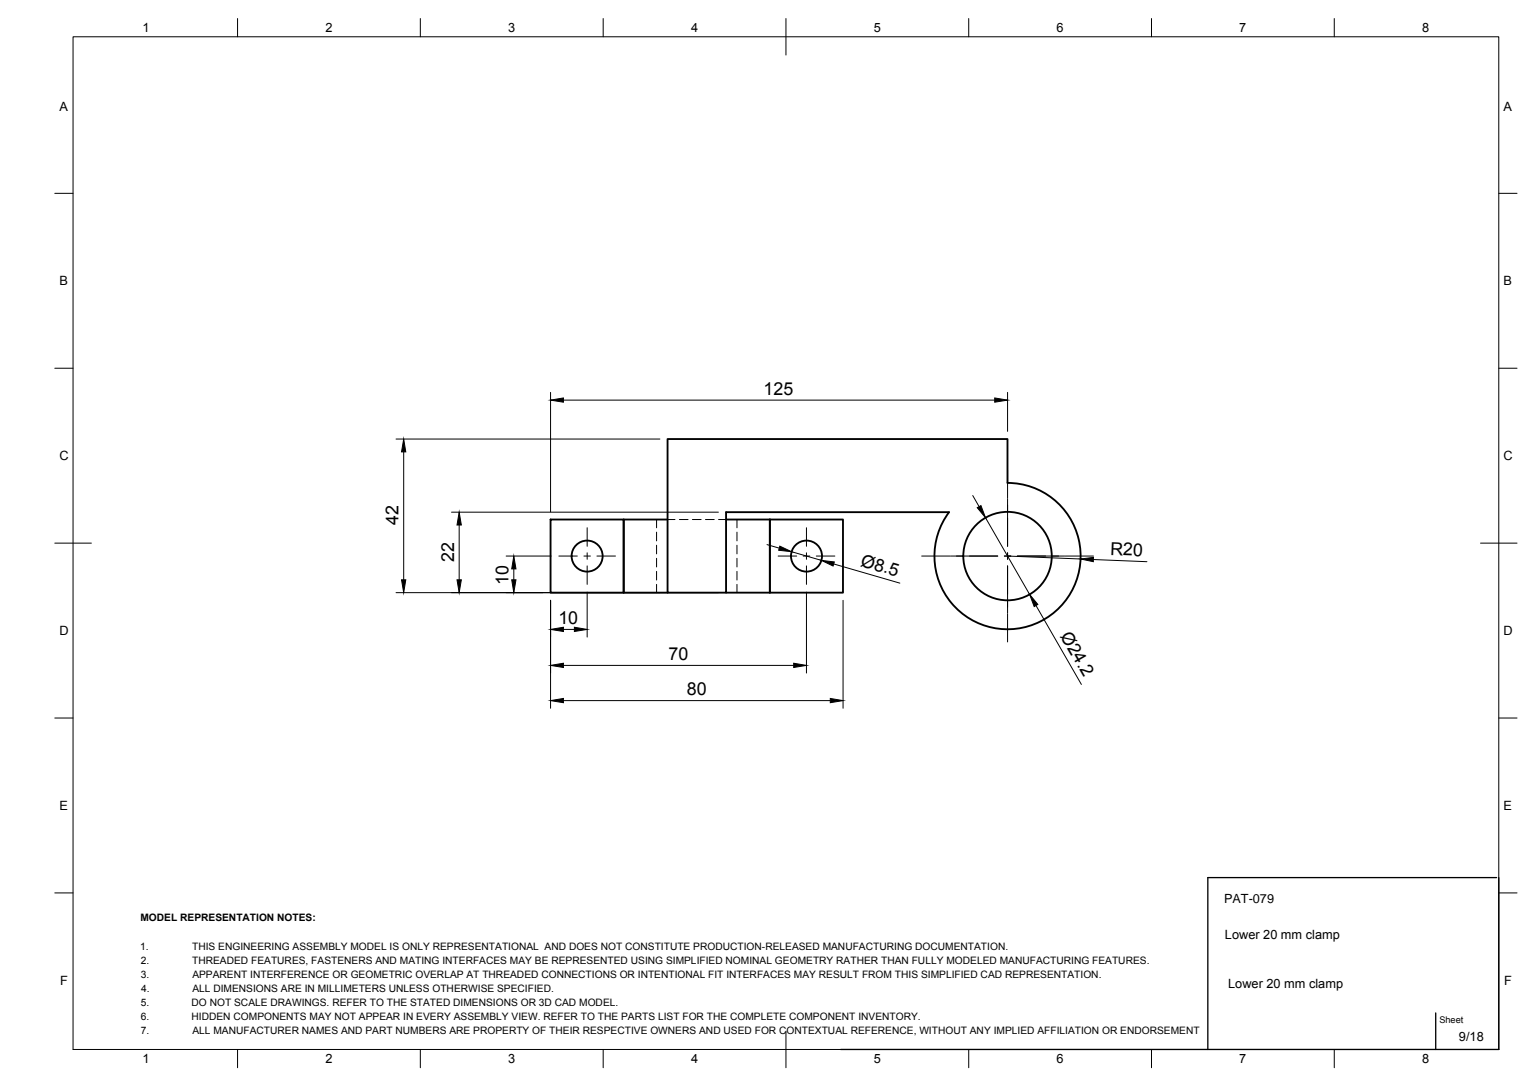
ISO-10303-21;
HEADER;
/* Generated by software containing ST-Developer
 * from STEP Tools, Inc. (www.steptools.com) 
 */

FILE_DESCRIPTION(
/* description */ ('Pipe clamp stand with threaded column'),
/* implementation_level */ '2;1');

FILE_NAME(
/* name */ 'Lower 20 mm clamp.step',
/* time_stamp */ '2026-10-27T10:55:48-07:00',
/* author */ (''),
/* organization */ (''),
/* preprocessor_version */ 'ST-DEVELOPER v20.2',
/* originating_system */ 'Autodesk Translation Framework v15.17.0.0',
/* authorisation */ '');

FILE_SCHEMA (('AUTOMOTIVE_DESIGN { 1 0 10303 214 3 1 1 }'));
ENDSEC;

DATA;
#10=MECHANICAL_DESIGN_GEOMETRIC_PRESENTATION_REPRESENTATION('',(#745,#746,#747),#34433);
#701=SHAPE_REPRESENTATION_RELATIONSHIP('SRR','None',#34543,#723);
#723=ADVANCED_BREP_SHAPE_REPRESENTATION('',(#775,#776,#777),#34411);
#745=STYLED_ITEM('',(#34729),#775);
#746=STYLED_ITEM('',(#34729),#776);
#747=STYLED_ITEM('',(#34729),#777);
#775=MANIFOLD_SOLID_BREP('Body1',#8772);
#776=MANIFOLD_SOLID_BREP('Body2',#8773);
#777=MANIFOLD_SOLID_BREP('Body3',#8774);
#822=FACE_BOUND('',#1783,.T.);
#823=FACE_BOUND('',#1787,.T.);
#824=FACE_BOUND('',#1797,.T.);
#825=FACE_BOUND('',#1800,.T.);
#826=FACE_BOUND('',#1806,.T.);
#827=FACE_BOUND('',#1809,.T.);
#872=PLANE('',#9307);
#873=PLANE('',#9310);
#874=PLANE('',#9317);
#875=PLANE('',#9318);
#876=PLANE('',#9319);
#877=PLANE('',#9320);
#878=PLANE('',#9321);
#879=PLANE('',#9322);
#880=PLANE('',#9323);
#881=PLANE('',#9324);
#882=PLANE('',#9329);
#883=PLANE('',#9333);
#884=PLANE('',#9334);
#885=PLANE('',#9335);
#886=PLANE('',#9336);
#887=PLANE('',#9337);
#888=PLANE('',#9338);
#889=PLANE('',#9342);
#890=PLANE('',#9343);
#891=PLANE('',#9344);
#892=PLANE('',#9345);
#893=PLANE('',#9346);
#894=PLANE('',#9347);
#1266=FACE_OUTER_BOUND('',#1776,.T.);
#1267=FACE_OUTER_BOUND('',#1777,.T.);
#1268=FACE_OUTER_BOUND('',#1778,.T.);
#1269=FACE_OUTER_BOUND('',#1779,.T.);
#1270=FACE_OUTER_BOUND('',#1780,.T.);
#1271=FACE_OUTER_BOUND('',#1781,.T.);
#1272=FACE_OUTER_BOUND('',#1782,.T.);
#1273=FACE_OUTER_BOUND('',#1784,.T.);
#1274=FACE_OUTER_BOUND('',#1785,.T.);
#1275=FACE_OUTER_BOUND('',#1786,.T.);
#1276=FACE_OUTER_BOUND('',#1788,.T.);
#1277=FACE_OUTER_BOUND('',#1789,.T.);
#1278=FACE_OUTER_BOUND('',#1790,.T.);
#1279=FACE_OUTER_BOUND('',#1791,.T.);
#1280=FACE_OUTER_BOUND('',#1792,.T.);
#1281=FACE_OUTER_BOUND('',#1793,.T.);
#1282=FACE_OUTER_BOUND('',#1794,.T.);
#1283=FACE_OUTER_BOUND('',#1795,.T.);
#1284=FACE_OUTER_BOUND('',#1796,.T.);
#1285=FACE_OUTER_BOUND('',#1798,.T.);
#1286=FACE_OUTER_BOUND('',#1799,.T.);
#1287=FACE_OUTER_BOUND('',#1801,.T.);
#1288=FACE_OUTER_BOUND('',#1802,.T.);
#1289=FACE_OUTER_BOUND('',#1803,.T.);
#1290=FACE_OUTER_BOUND('',#1804,.T.);
#1291=FACE_OUTER_BOUND('',#1805,.T.);
#1292=FACE_OUTER_BOUND('',#1807,.T.);
#1293=FACE_OUTER_BOUND('',#1808,.T.);
#1294=FACE_OUTER_BOUND('',#1810,.T.);
#1295=FACE_OUTER_BOUND('',#1811,.T.);
#1776=EDGE_LOOP('',(#6779,#6780,#6781,#6782));
#1777=EDGE_LOOP('',(#6783,#6784,#6785,#6786,#6787,#6788,#6789,#6790));
#1778=EDGE_LOOP('',(#6791,#6792,#6793,#6794));
#1779=EDGE_LOOP('',(#6795,#6796,#6797,#6798));
#1780=EDGE_LOOP('',(#6799,#6800,#6801,#6802));
#1781=EDGE_LOOP('',(#6803,#6804,#6805,#6806));
#1782=EDGE_LOOP('',(#6807,#6808,#6809,#6810,#6811,#6812,#6813));
#1783=EDGE_LOOP('',(#6814));
#1784=EDGE_LOOP('',(#6815,#6816,#6817,#6818));
#1785=EDGE_LOOP('',(#6819,#6820,#6821,#6822));
#1786=EDGE_LOOP('',(#6823,#6824,#6825,#6826,#6827,#6828,#6829));
#1787=EDGE_LOOP('',(#6830));
#1788=EDGE_LOOP('',(#6831,#6832,#6833,#6834,#6835,#6836));
#1789=EDGE_LOOP('',(#6837,#6838,#6839,#6840,#6841,#6842));
#1790=EDGE_LOOP('',(#6843,#6844,#6845,#6846,#6847,#6848,#6849,#6850));
#1791=EDGE_LOOP('',(#6851,#6852,#6853,#6854));
#1792=EDGE_LOOP('',(#6855,#6856,#6857,#6858));
#1793=EDGE_LOOP('',(#6859,#6860,#6861,#6862));
#1794=EDGE_LOOP('',(#6863,#6864,#6865,#6866));
#1795=EDGE_LOOP('',(#6867,#6868,#6869,#6870));
#1796=EDGE_LOOP('',(#6871,#6872,#6873,#6874));
#1797=EDGE_LOOP('',(#6875));
#1798=EDGE_LOOP('',(#6876,#6877,#6878,#6879));
#1799=EDGE_LOOP('',(#6880,#6881,#6882,#6883));
#1800=EDGE_LOOP('',(#6884));
#1801=EDGE_LOOP('',(#6885,#6886,#6887,#6888));
#1802=EDGE_LOOP('',(#6889,#6890,#6891,#6892));
#1803=EDGE_LOOP('',(#6893,#6894,#6895,#6896));
#1804=EDGE_LOOP('',(#6897,#6898,#6899,#6900));
#1805=EDGE_LOOP('',(#6901,#6902,#6903,#6904));
#1806=EDGE_LOOP('',(#6905));
#1807=EDGE_LOOP('',(#6906,#6907,#6908,#6909));
#1808=EDGE_LOOP('',(#6910,#6911,#6912,#6913));
#1809=EDGE_LOOP('',(#6914));
#1810=EDGE_LOOP('',(#6915,#6916,#6917,#6918));
#1811=EDGE_LOOP('',(#6919,#6920,#6921,#6922));
#2291=LINE('',#28038,#2908);
#2292=LINE('',#28041,#2909);
#2293=LINE('',#28044,#2910);
#2294=LINE('',#28048,#2911);
#2295=LINE('',#28050,#2912);
#2296=LINE('',#28052,#2913);
#2297=LINE('',#28055,#2914);
#2298=LINE('',#28058,#2915);
#2299=LINE('',#28059,#2916);
#2300=LINE('',#28064,#2917);
#2301=LINE('',#28069,#2918);
#2302=LINE('',#28073,#2919);
#2303=LINE('',#28077,#2920);
#2304=LINE('',#28079,#2921);
#2305=LINE('',#28080,#2922);
#2306=LINE('',#28083,#2923);
#2307=LINE('',#28085,#2924);
#2308=LINE('',#28087,#2925);
#2309=LINE('',#28089,#2926);
#2310=LINE('',#28090,#2927);
#2311=LINE('',#28093,#2928);
#2312=LINE('',#28094,#2929);
#2313=LINE('',#28097,#2930);
#2314=LINE('',#28098,#2931);
#2315=LINE('',#28100,#2932);
#2316=LINE('',#28101,#2933);
#2317=LINE('',#28104,#2934);
#2318=LINE('',#28105,#2935);
#2319=LINE('',#28108,#2936);
#2320=LINE('',#28109,#2937);
#2321=LINE('',#28112,#2938);
#2322=LINE('',#28117,#2939);
#2323=LINE('',#28123,#2940);
#2324=LINE('',#28128,#2941);
#2325=LINE('',#28130,#2942);
#2326=LINE('',#28132,#2943);
#2327=LINE('',#28133,#2944);
#2328=LINE('',#28136,#2945);
#2329=LINE('',#28138,#2946);
#2330=LINE('',#28139,#2947);
#2331=LINE('',#28142,#2948);
#2332=LINE('',#28144,#2949);
#2333=LINE('',#28145,#2950);
#2334=LINE('',#28147,#2951);
#2335=LINE('',#28148,#2952);
#2336=LINE('',#28155,#2953);
#2337=LINE('',#28160,#2954);
#2338=LINE('',#28162,#2955);
#2339=LINE('',#28164,#2956);
#2340=LINE('',#28165,#2957);
#2341=LINE('',#28168,#2958);
#2342=LINE('',#28170,#2959);
#2343=LINE('',#28171,#2960);
#2344=LINE('',#28174,#2961);
#2345=LINE('',#28176,#2962);
#2346=LINE('',#28177,#2963);
#2347=LINE('',#28179,#2964);
#2348=LINE('',#28180,#2965);
#2908=VECTOR('',#10466,1.);
#2909=VECTOR('',#10469,1.);
#2910=VECTOR('',#10472,1.);
#2911=VECTOR('',#10475,1.);
#2912=VECTOR('',#10476,1.);
#2913=VECTOR('',#10477,1.);
#2914=VECTOR('',#10480,1.);
#2915=VECTOR('',#10483,1.);
#2916=VECTOR('',#10484,1.);
#2917=VECTOR('',#10489,1.21);
#2918=VECTOR('',#10494,1.);
#2919=VECTOR('',#10497,1.);
#2920=VECTOR('',#10502,1.);
#2921=VECTOR('',#10503,1.);
#2922=VECTOR('',#10504,1.);
#2923=VECTOR('',#10507,1.);
#2924=VECTOR('',#10508,1.);
#2925=VECTOR('',#10509,1.);
#2926=VECTOR('',#10510,1.);
#2927=VECTOR('',#10511,1.);
#2928=VECTOR('',#10514,1.);
#2929=VECTOR('',#10515,1.);
#2930=VECTOR('',#10518,1.);
#2931=VECTOR('',#10519,1.);
#2932=VECTOR('',#10522,1.);
#2933=VECTOR('',#10523,1.);
#2934=VECTOR('',#10526,1.);
#2935=VECTOR('',#10527,1.);
#2936=VECTOR('',#10530,1.);
#2937=VECTOR('',#10531,1.);
#2938=VECTOR('',#10534,1.);
#2939=VECTOR('',#10543,1.);
#2940=VECTOR('',#10550,0.425);
#2941=VECTOR('',#10555,1.);
#2942=VECTOR('',#10556,1.);
#2943=VECTOR('',#10557,1.);
#2944=VECTOR('',#10558,1.);
#2945=VECTOR('',#10561,1.);
#2946=VECTOR('',#10562,1.);
#2947=VECTOR('',#10563,1.);
#2948=VECTOR('',#10566,1.);
#2949=VECTOR('',#10567,1.);
#2950=VECTOR('',#10568,1.);
#2951=VECTOR('',#10571,1.);
#2952=VECTOR('',#10572,1.);
#2953=VECTOR('',#10581,0.425);
#2954=VECTOR('',#10586,1.);
#2955=VECTOR('',#10587,1.);
#2956=VECTOR('',#10588,1.);
#2957=VECTOR('',#10589,1.);
#2958=VECTOR('',#10592,1.);
#2959=VECTOR('',#10593,1.);
#2960=VECTOR('',#10594,1.);
#2961=VECTOR('',#10597,1.);
#2962=VECTOR('',#10598,1.);
#2963=VECTOR('',#10599,1.);
#2964=VECTOR('',#10602,1.);
#2965=VECTOR('',#10603,1.);
#3344=CIRCLE('',#9305,1.1);
#3345=CIRCLE('',#9306,1.1);
#3346=CIRCLE('',#9308,2.);
#3347=CIRCLE('',#9309,2.);
#3348=CIRCLE('',#9312,1.21);
#3349=CIRCLE('',#9313,1.21);
#3350=CIRCLE('',#9315,2.);
#3351=CIRCLE('',#9316,2.);
#3352=CIRCLE('',#9325,2.);
#3353=CIRCLE('',#9326,2.);
#3354=CIRCLE('',#9331,0.425);
#3355=CIRCLE('',#9332,0.425);
#3356=CIRCLE('',#9340,0.425);
#3357=CIRCLE('',#9341,0.425);
#3866=VERTEX_POINT('',#28034);
#3867=VERTEX_POINT('',#28035);
#3868=VERTEX_POINT('',#28037);
#3869=VERTEX_POINT('',#28039);
#3870=VERTEX_POINT('',#28043);
#3871=VERTEX_POINT('',#28045);
#3872=VERTEX_POINT('',#28047);
#3873=VERTEX_POINT('',#28049);
#3874=VERTEX_POINT('',#28051);
#3875=VERTEX_POINT('',#28053);
#3876=VERTEX_POINT('',#28057);
#3877=VERTEX_POINT('',#28061);
#3878=VERTEX_POINT('',#28063);
#3879=VERTEX_POINT('',#28067);
#3880=VERTEX_POINT('',#28068);
#3881=VERTEX_POINT('',#28070);
#3882=VERTEX_POINT('',#28072);
#3883=VERTEX_POINT('',#28076);
#3884=VERTEX_POINT('',#28078);
#3885=VERTEX_POINT('',#28082);
#3886=VERTEX_POINT('',#28084);
#3887=VERTEX_POINT('',#28086);
#3888=VERTEX_POINT('',#28088);
#3889=VERTEX_POINT('',#28092);
#3890=VERTEX_POINT('',#28096);
#3891=VERTEX_POINT('',#28103);
#3892=VERTEX_POINT('',#28107);
#3893=VERTEX_POINT('',#28111);
#3894=VERTEX_POINT('',#28120);
#3895=VERTEX_POINT('',#28122);
#3896=VERTEX_POINT('',#28126);
#3897=VERTEX_POINT('',#28127);
#3898=VERTEX_POINT('',#28129);
#3899=VERTEX_POINT('',#28131);
#3900=VERTEX_POINT('',#28135);
#3901=VERTEX_POINT('',#28137);
#3902=VERTEX_POINT('',#28141);
#3903=VERTEX_POINT('',#28143);
#3904=VERTEX_POINT('',#28152);
#3905=VERTEX_POINT('',#28154);
#3906=VERTEX_POINT('',#28158);
#3907=VERTEX_POINT('',#28159);
#3908=VERTEX_POINT('',#28161);
#3909=VERTEX_POINT('',#28163);
#3910=VERTEX_POINT('',#28167);
#3911=VERTEX_POINT('',#28169);
#3912=VERTEX_POINT('',#28173);
#3913=VERTEX_POINT('',#28175);
#4903=EDGE_CURVE('',#3866,#3867,#3344,.T.);
#4904=EDGE_CURVE('',#3868,#3866,#2291,.T.);
#4905=EDGE_CURVE('',#3869,#3868,#3345,.T.);
#4906=EDGE_CURVE('',#3867,#3869,#2292,.T.);
#4907=EDGE_CURVE('',#3868,#3870,#2293,.T.);
#4908=EDGE_CURVE('',#3870,#3871,#3346,.T.);
#4909=EDGE_CURVE('',#3871,#3872,#2294,.T.);
#4910=EDGE_CURVE('',#3872,#3873,#2295,.T.);
#4911=EDGE_CURVE('',#3873,#3874,#2296,.T.);
#4912=EDGE_CURVE('',#3874,#3875,#3347,.T.);
#4913=EDGE_CURVE('',#3875,#3869,#2297,.T.);
#4914=EDGE_CURVE('',#3876,#3866,#2298,.T.);
#4915=EDGE_CURVE('',#3870,#3876,#2299,.T.);
#4916=EDGE_CURVE('',#3877,#3877,#3348,.T.);
#4917=EDGE_CURVE('',#3877,#3878,#2300,.T.);
#4918=EDGE_CURVE('',#3878,#3878,#3349,.T.);
#4919=EDGE_CURVE('',#3879,#3880,#2301,.T.);
#4920=EDGE_CURVE('',#3881,#3879,#3350,.T.);
#4921=EDGE_CURVE('',#3882,#3881,#2302,.T.);
#4922=EDGE_CURVE('',#3882,#3880,#3351,.T.);
#4923=EDGE_CURVE('',#3880,#3883,#2303,.T.);
#4924=EDGE_CURVE('',#3884,#3883,#2304,.T.);
#4925=EDGE_CURVE('',#3884,#3879,#2305,.T.);
#4926=EDGE_CURVE('',#3882,#3885,#2306,.T.);
#4927=EDGE_CURVE('',#3886,#3885,#2307,.T.);
#4928=EDGE_CURVE('',#3887,#3886,#2308,.T.);
#4929=EDGE_CURVE('',#3888,#3887,#2309,.T.);
#4930=EDGE_CURVE('',#3888,#3883,#2310,.T.);
#4931=EDGE_CURVE('',#3881,#3889,#2311,.T.);
#4932=EDGE_CURVE('',#3885,#3889,#2312,.T.);
#4933=EDGE_CURVE('',#3889,#3890,#2313,.T.);
#4934=EDGE_CURVE('',#3890,#3886,#2314,.T.);
#4935=EDGE_CURVE('',#3873,#3884,#2315,.T.);
#4936=EDGE_CURVE('',#3872,#3890,#2316,.T.);
#4937=EDGE_CURVE('',#3891,#3888,#2317,.T.);
#4938=EDGE_CURVE('',#3874,#3891,#2318,.T.);
#4939=EDGE_CURVE('',#3892,#3871,#2319,.T.);
#4940=EDGE_CURVE('',#3887,#3892,#2320,.T.);
#4941=EDGE_CURVE('',#3867,#3893,#2321,.T.);
#4942=EDGE_CURVE('',#3891,#3893,#3352,.T.);
#4943=EDGE_CURVE('',#3876,#3892,#3353,.T.);
#4944=EDGE_CURVE('',#3893,#3875,#2322,.T.);
#4945=EDGE_CURVE('',#3894,#3894,#3354,.T.);
#4946=EDGE_CURVE('',#3894,#3895,#2323,.T.);
#4947=EDGE_CURVE('',#3895,#3895,#3355,.T.);
#4948=EDGE_CURVE('',#3896,#3897,#2324,.T.);
#4949=EDGE_CURVE('',#3896,#3898,#2325,.T.);
#4950=EDGE_CURVE('',#3899,#3898,#2326,.T.);
#4951=EDGE_CURVE('',#3897,#3899,#2327,.T.);
#4952=EDGE_CURVE('',#3897,#3900,#2328,.T.);
#4953=EDGE_CURVE('',#3901,#3899,#2329,.T.);
#4954=EDGE_CURVE('',#3900,#3901,#2330,.T.);
#4955=EDGE_CURVE('',#3900,#3902,#2331,.T.);
#4956=EDGE_CURVE('',#3903,#3901,#2332,.T.);
#4957=EDGE_CURVE('',#3902,#3903,#2333,.T.);
#4958=EDGE_CURVE('',#3902,#3896,#2334,.T.);
#4959=EDGE_CURVE('',#3898,#3903,#2335,.T.);
#4960=EDGE_CURVE('',#3904,#3904,#3356,.T.);
#4961=EDGE_CURVE('',#3904,#3905,#2336,.T.);
#4962=EDGE_CURVE('',#3905,#3905,#3357,.T.);
#4963=EDGE_CURVE('',#3906,#3907,#2337,.T.);
#4964=EDGE_CURVE('',#3906,#3908,#2338,.T.);
#4965=EDGE_CURVE('',#3909,#3908,#2339,.T.);
#4966=EDGE_CURVE('',#3907,#3909,#2340,.T.);
#4967=EDGE_CURVE('',#3907,#3910,#2341,.T.);
#4968=EDGE_CURVE('',#3911,#3909,#2342,.T.);
#4969=EDGE_CURVE('',#3910,#3911,#2343,.T.);
#4970=EDGE_CURVE('',#3910,#3912,#2344,.T.);
#4971=EDGE_CURVE('',#3913,#3911,#2345,.T.);
#4972=EDGE_CURVE('',#3912,#3913,#2346,.T.);
#4973=EDGE_CURVE('',#3912,#3906,#2347,.T.);
#4974=EDGE_CURVE('',#3908,#3913,#2348,.T.);
#6779=ORIENTED_EDGE('',*,*,#4903,.F.);
#6780=ORIENTED_EDGE('',*,*,#4904,.F.);
#6781=ORIENTED_EDGE('',*,*,#4905,.F.);
#6782=ORIENTED_EDGE('',*,*,#4906,.F.);
#6783=ORIENTED_EDGE('',*,*,#4905,.T.);
#6784=ORIENTED_EDGE('',*,*,#4907,.T.);
#6785=ORIENTED_EDGE('',*,*,#4908,.T.);
#6786=ORIENTED_EDGE('',*,*,#4909,.T.);
#6787=ORIENTED_EDGE('',*,*,#4910,.T.);
#6788=ORIENTED_EDGE('',*,*,#4911,.T.);
#6789=ORIENTED_EDGE('',*,*,#4912,.T.);
#6790=ORIENTED_EDGE('',*,*,#4913,.T.);
#6791=ORIENTED_EDGE('',*,*,#4904,.T.);
#6792=ORIENTED_EDGE('',*,*,#4914,.F.);
#6793=ORIENTED_EDGE('',*,*,#4915,.F.);
#6794=ORIENTED_EDGE('',*,*,#4907,.F.);
#6795=ORIENTED_EDGE('',*,*,#4916,.F.);
#6796=ORIENTED_EDGE('',*,*,#4917,.T.);
#6797=ORIENTED_EDGE('',*,*,#4918,.F.);
#6798=ORIENTED_EDGE('',*,*,#4917,.F.);
#6799=ORIENTED_EDGE('',*,*,#4919,.F.);
#6800=ORIENTED_EDGE('',*,*,#4920,.F.);
#6801=ORIENTED_EDGE('',*,*,#4921,.F.);
#6802=ORIENTED_EDGE('',*,*,#4922,.T.);
#6803=ORIENTED_EDGE('',*,*,#4919,.T.);
#6804=ORIENTED_EDGE('',*,*,#4923,.T.);
#6805=ORIENTED_EDGE('',*,*,#4924,.F.);
#6806=ORIENTED_EDGE('',*,*,#4925,.T.);
#6807=ORIENTED_EDGE('',*,*,#4926,.T.);
#6808=ORIENTED_EDGE('',*,*,#4927,.F.);
#6809=ORIENTED_EDGE('',*,*,#4928,.F.);
#6810=ORIENTED_EDGE('',*,*,#4929,.F.);
#6811=ORIENTED_EDGE('',*,*,#4930,.T.);
#6812=ORIENTED_EDGE('',*,*,#4923,.F.);
#6813=ORIENTED_EDGE('',*,*,#4922,.F.);
#6814=ORIENTED_EDGE('',*,*,#4916,.T.);
#6815=ORIENTED_EDGE('',*,*,#4921,.T.);
#6816=ORIENTED_EDGE('',*,*,#4931,.T.);
#6817=ORIENTED_EDGE('',*,*,#4932,.F.);
#6818=ORIENTED_EDGE('',*,*,#4926,.F.);
#6819=ORIENTED_EDGE('',*,*,#4933,.T.);
#6820=ORIENTED_EDGE('',*,*,#4934,.T.);
#6821=ORIENTED_EDGE('',*,*,#4927,.T.);
#6822=ORIENTED_EDGE('',*,*,#4932,.T.);
#6823=ORIENTED_EDGE('',*,*,#4925,.F.);
#6824=ORIENTED_EDGE('',*,*,#4935,.F.);
#6825=ORIENTED_EDGE('',*,*,#4910,.F.);
#6826=ORIENTED_EDGE('',*,*,#4936,.T.);
#6827=ORIENTED_EDGE('',*,*,#4933,.F.);
#6828=ORIENTED_EDGE('',*,*,#4931,.F.);
#6829=ORIENTED_EDGE('',*,*,#4920,.T.);
#6830=ORIENTED_EDGE('',*,*,#4918,.T.);
#6831=ORIENTED_EDGE('',*,*,#4924,.T.);
#6832=ORIENTED_EDGE('',*,*,#4930,.F.);
#6833=ORIENTED_EDGE('',*,*,#4937,.F.);
#6834=ORIENTED_EDGE('',*,*,#4938,.F.);
#6835=ORIENTED_EDGE('',*,*,#4911,.F.);
#6836=ORIENTED_EDGE('',*,*,#4935,.T.);
#6837=ORIENTED_EDGE('',*,*,#4939,.F.);
#6838=ORIENTED_EDGE('',*,*,#4940,.F.);
#6839=ORIENTED_EDGE('',*,*,#4928,.T.);
#6840=ORIENTED_EDGE('',*,*,#4934,.F.);
#6841=ORIENTED_EDGE('',*,*,#4936,.F.);
#6842=ORIENTED_EDGE('',*,*,#4909,.F.);
#6843=ORIENTED_EDGE('',*,*,#4903,.T.);
#6844=ORIENTED_EDGE('',*,*,#4941,.T.);
#6845=ORIENTED_EDGE('',*,*,#4942,.F.);
#6846=ORIENTED_EDGE('',*,*,#4937,.T.);
#6847=ORIENTED_EDGE('',*,*,#4929,.T.);
#6848=ORIENTED_EDGE('',*,*,#4940,.T.);
#6849=ORIENTED_EDGE('',*,*,#4943,.F.);
#6850=ORIENTED_EDGE('',*,*,#4914,.T.);
#6851=ORIENTED_EDGE('',*,*,#4939,.T.);
#6852=ORIENTED_EDGE('',*,*,#4908,.F.);
#6853=ORIENTED_EDGE('',*,*,#4915,.T.);
#6854=ORIENTED_EDGE('',*,*,#4943,.T.);
#6855=ORIENTED_EDGE('',*,*,#4938,.T.);
#6856=ORIENTED_EDGE('',*,*,#4942,.T.);
#6857=ORIENTED_EDGE('',*,*,#4944,.T.);
#6858=ORIENTED_EDGE('',*,*,#4912,.F.);
#6859=ORIENTED_EDGE('',*,*,#4906,.T.);
#6860=ORIENTED_EDGE('',*,*,#4913,.F.);
#6861=ORIENTED_EDGE('',*,*,#4944,.F.);
#6862=ORIENTED_EDGE('',*,*,#4941,.F.);
#6863=ORIENTED_EDGE('',*,*,#4945,.F.);
#6864=ORIENTED_EDGE('',*,*,#4946,.T.);
#6865=ORIENTED_EDGE('',*,*,#4947,.F.);
#6866=ORIENTED_EDGE('',*,*,#4946,.F.);
#6867=ORIENTED_EDGE('',*,*,#4948,.F.);
#6868=ORIENTED_EDGE('',*,*,#4949,.T.);
#6869=ORIENTED_EDGE('',*,*,#4950,.F.);
#6870=ORIENTED_EDGE('',*,*,#4951,.F.);
#6871=ORIENTED_EDGE('',*,*,#4952,.F.);
#6872=ORIENTED_EDGE('',*,*,#4951,.T.);
#6873=ORIENTED_EDGE('',*,*,#4953,.F.);
#6874=ORIENTED_EDGE('',*,*,#4954,.F.);
#6875=ORIENTED_EDGE('',*,*,#4945,.T.);
#6876=ORIENTED_EDGE('',*,*,#4955,.F.);
#6877=ORIENTED_EDGE('',*,*,#4954,.T.);
#6878=ORIENTED_EDGE('',*,*,#4956,.F.);
#6879=ORIENTED_EDGE('',*,*,#4957,.F.);
#6880=ORIENTED_EDGE('',*,*,#4958,.F.);
#6881=ORIENTED_EDGE('',*,*,#4957,.T.);
#6882=ORIENTED_EDGE('',*,*,#4959,.F.);
#6883=ORIENTED_EDGE('',*,*,#4949,.F.);
#6884=ORIENTED_EDGE('',*,*,#4947,.T.);
#6885=ORIENTED_EDGE('',*,*,#4959,.T.);
#6886=ORIENTED_EDGE('',*,*,#4956,.T.);
#6887=ORIENTED_EDGE('',*,*,#4953,.T.);
#6888=ORIENTED_EDGE('',*,*,#4950,.T.);
#6889=ORIENTED_EDGE('',*,*,#4958,.T.);
#6890=ORIENTED_EDGE('',*,*,#4948,.T.);
#6891=ORIENTED_EDGE('',*,*,#4952,.T.);
#6892=ORIENTED_EDGE('',*,*,#4955,.T.);
#6893=ORIENTED_EDGE('',*,*,#4960,.F.);
#6894=ORIENTED_EDGE('',*,*,#4961,.T.);
#6895=ORIENTED_EDGE('',*,*,#4962,.F.);
#6896=ORIENTED_EDGE('',*,*,#4961,.F.);
#6897=ORIENTED_EDGE('',*,*,#4963,.F.);
#6898=ORIENTED_EDGE('',*,*,#4964,.T.);
#6899=ORIENTED_EDGE('',*,*,#4965,.F.);
#6900=ORIENTED_EDGE('',*,*,#4966,.F.);
#6901=ORIENTED_EDGE('',*,*,#4967,.F.);
#6902=ORIENTED_EDGE('',*,*,#4966,.T.);
#6903=ORIENTED_EDGE('',*,*,#4968,.F.);
#6904=ORIENTED_EDGE('',*,*,#4969,.F.);
#6905=ORIENTED_EDGE('',*,*,#4960,.T.);
#6906=ORIENTED_EDGE('',*,*,#4970,.F.);
#6907=ORIENTED_EDGE('',*,*,#4969,.T.);
#6908=ORIENTED_EDGE('',*,*,#4971,.F.);
#6909=ORIENTED_EDGE('',*,*,#4972,.F.);
#6910=ORIENTED_EDGE('',*,*,#4973,.F.);
#6911=ORIENTED_EDGE('',*,*,#4972,.T.);
#6912=ORIENTED_EDGE('',*,*,#4974,.F.);
#6913=ORIENTED_EDGE('',*,*,#4964,.F.);
#6914=ORIENTED_EDGE('',*,*,#4962,.T.);
#6915=ORIENTED_EDGE('',*,*,#4974,.T.);
#6916=ORIENTED_EDGE('',*,*,#4971,.T.);
#6917=ORIENTED_EDGE('',*,*,#4968,.T.);
#6918=ORIENTED_EDGE('',*,*,#4965,.T.);
#6919=ORIENTED_EDGE('',*,*,#4973,.T.);
#6920=ORIENTED_EDGE('',*,*,#4963,.T.);
#6921=ORIENTED_EDGE('',*,*,#4967,.T.);
#6922=ORIENTED_EDGE('',*,*,#4970,.T.);
#8204=CYLINDRICAL_SURFACE('',#9304,1.1);
#8205=CYLINDRICAL_SURFACE('',#9311,1.21);
#8206=CYLINDRICAL_SURFACE('',#9314,2.);
#8207=CYLINDRICAL_SURFACE('',#9327,2.);
#8208=CYLINDRICAL_SURFACE('',#9328,2.);
#8209=CYLINDRICAL_SURFACE('',#9330,0.425);
#8210=CYLINDRICAL_SURFACE('',#9339,0.425);
#8503=ADVANCED_FACE('',(#1266),#8204,.F.);
#8504=ADVANCED_FACE('',(#1267),#872,.T.);
#8505=ADVANCED_FACE('',(#1268),#873,.F.);
#8506=ADVANCED_FACE('',(#1269),#8205,.F.);
#8507=ADVANCED_FACE('',(#1270),#8206,.T.);
#8508=ADVANCED_FACE('',(#1271),#874,.F.);
#8509=ADVANCED_FACE('',(#1272,#822),#875,.T.);
#8510=ADVANCED_FACE('',(#1273),#876,.T.);
#8511=ADVANCED_FACE('',(#1274),#877,.T.);
#8512=ADVANCED_FACE('',(#1275,#823),#878,.T.);
#8513=ADVANCED_FACE('',(#1276),#879,.T.);
#8514=ADVANCED_FACE('',(#1277),#880,.T.);
#8515=ADVANCED_FACE('',(#1278),#881,.F.);
#8516=ADVANCED_FACE('',(#1279),#8207,.T.);
#8517=ADVANCED_FACE('',(#1280),#8208,.T.);
#8518=ADVANCED_FACE('',(#1281),#882,.F.);
#8519=ADVANCED_FACE('',(#1282),#8209,.F.);
#8520=ADVANCED_FACE('',(#1283),#883,.T.);
#8521=ADVANCED_FACE('',(#1284,#824),#884,.T.);
#8522=ADVANCED_FACE('',(#1285),#885,.T.);
#8523=ADVANCED_FACE('',(#1286,#825),#886,.T.);
#8524=ADVANCED_FACE('',(#1287),#887,.T.);
#8525=ADVANCED_FACE('',(#1288),#888,.F.);
#8526=ADVANCED_FACE('',(#1289),#8210,.F.);
#8527=ADVANCED_FACE('',(#1290),#889,.T.);
#8528=ADVANCED_FACE('',(#1291,#826),#890,.T.);
#8529=ADVANCED_FACE('',(#1292),#891,.T.);
#8530=ADVANCED_FACE('',(#1293,#827),#892,.T.);
#8531=ADVANCED_FACE('',(#1294),#893,.T.);
#8532=ADVANCED_FACE('',(#1295),#894,.F.);
#8772=CLOSED_SHELL('',(#8503,#8504,#8505,#8506,#8507,#8508,#8509,#8510,
#8511,#8512,#8513,#8514,#8515,#8516,#8517,#8518));
#8773=CLOSED_SHELL('',(#8519,#8520,#8521,#8522,#8523,#8524,#8525));
#8774=CLOSED_SHELL('',(#8526,#8527,#8528,#8529,#8530,#8531,#8532));
#9303=AXIS2_PLACEMENT_3D('',#28032,#10460,#10461);
#9304=AXIS2_PLACEMENT_3D('',#28033,#10462,#10463);
#9305=AXIS2_PLACEMENT_3D('',#28036,#10464,#10465);
#9306=AXIS2_PLACEMENT_3D('',#28040,#10467,#10468);
#9307=AXIS2_PLACEMENT_3D('',#28042,#10470,#10471);
#9308=AXIS2_PLACEMENT_3D('',#28046,#10473,#10474);
#9309=AXIS2_PLACEMENT_3D('',#28054,#10478,#10479);
#9310=AXIS2_PLACEMENT_3D('',#28056,#10481,#10482);
#9311=AXIS2_PLACEMENT_3D('',#28060,#10485,#10486);
#9312=AXIS2_PLACEMENT_3D('',#28062,#10487,#10488);
#9313=AXIS2_PLACEMENT_3D('',#28065,#10490,#10491);
#9314=AXIS2_PLACEMENT_3D('',#28066,#10492,#10493);
#9315=AXIS2_PLACEMENT_3D('',#28071,#10495,#10496);
#9316=AXIS2_PLACEMENT_3D('',#28074,#10498,#10499);
#9317=AXIS2_PLACEMENT_3D('',#28075,#10500,#10501);
#9318=AXIS2_PLACEMENT_3D('',#28081,#10505,#10506);
#9319=AXIS2_PLACEMENT_3D('',#28091,#10512,#10513);
#9320=AXIS2_PLACEMENT_3D('',#28095,#10516,#10517);
#9321=AXIS2_PLACEMENT_3D('',#28099,#10520,#10521);
#9322=AXIS2_PLACEMENT_3D('',#28102,#10524,#10525);
#9323=AXIS2_PLACEMENT_3D('',#28106,#10528,#10529);
#9324=AXIS2_PLACEMENT_3D('',#28110,#10532,#10533);
#9325=AXIS2_PLACEMENT_3D('',#28113,#10535,#10536);
#9326=AXIS2_PLACEMENT_3D('',#28114,#10537,#10538);
#9327=AXIS2_PLACEMENT_3D('',#28115,#10539,#10540);
#9328=AXIS2_PLACEMENT_3D('',#28116,#10541,#10542);
#9329=AXIS2_PLACEMENT_3D('',#28118,#10544,#10545);
#9330=AXIS2_PLACEMENT_3D('',#28119,#10546,#10547);
#9331=AXIS2_PLACEMENT_3D('',#28121,#10548,#10549);
#9332=AXIS2_PLACEMENT_3D('',#28124,#10551,#10552);
#9333=AXIS2_PLACEMENT_3D('',#28125,#10553,#10554);
#9334=AXIS2_PLACEMENT_3D('',#28134,#10559,#10560);
#9335=AXIS2_PLACEMENT_3D('',#28140,#10564,#10565);
#9336=AXIS2_PLACEMENT_3D('',#28146,#10569,#10570);
#9337=AXIS2_PLACEMENT_3D('',#28149,#10573,#10574);
#9338=AXIS2_PLACEMENT_3D('',#28150,#10575,#10576);
#9339=AXIS2_PLACEMENT_3D('',#28151,#10577,#10578);
#9340=AXIS2_PLACEMENT_3D('',#28153,#10579,#10580);
#9341=AXIS2_PLACEMENT_3D('',#28156,#10582,#10583);
#9342=AXIS2_PLACEMENT_3D('',#28157,#10584,#10585);
#9343=AXIS2_PLACEMENT_3D('',#28166,#10590,#10591);
#9344=AXIS2_PLACEMENT_3D('',#28172,#10595,#10596);
#9345=AXIS2_PLACEMENT_3D('',#28178,#10600,#10601);
#9346=AXIS2_PLACEMENT_3D('',#28181,#10604,#10605);
#9347=AXIS2_PLACEMENT_3D('',#28182,#10606,#10607);
#10460=DIRECTION('axis',(0.,0.,1.));
#10461=DIRECTION('refdir',(1.,0.,0.));
#10462=DIRECTION('center_axis',(0.,1.,0.));
#10463=DIRECTION('ref_axis',(1.,0.,0.));
#10464=DIRECTION('center_axis',(0.,1.,0.));
#10465=DIRECTION('ref_axis',(1.,0.,0.));
#10466=DIRECTION('',(0.,-1.,0.));
#10467=DIRECTION('center_axis',(0.,-1.,0.));
#10468=DIRECTION('ref_axis',(1.,0.,0.));
#10469=DIRECTION('',(0.,1.,0.));
#10470=DIRECTION('center_axis',(0.,1.,0.));
#10471=DIRECTION('ref_axis',(1.,0.,0.));
#10472=DIRECTION('',(1.,0.,0.));
#10473=DIRECTION('center_axis',(0.,1.,0.));
#10474=DIRECTION('ref_axis',(1.,0.,0.));
#10475=DIRECTION('',(0.,0.,1.));
#10476=DIRECTION('',(-1.,0.,0.));
#10477=DIRECTION('',(0.,0.,-1.));
#10478=DIRECTION('center_axis',(0.,1.,0.));
#10479=DIRECTION('ref_axis',(1.,0.,0.));
#10480=DIRECTION('',(1.,0.,0.));
#10481=DIRECTION('center_axis',(0.,0.,-1.));
#10482=DIRECTION('ref_axis',(-1.,0.,0.));
#10483=DIRECTION('',(-1.,0.,0.));
#10484=DIRECTION('',(0.,-1.,0.));
#10485=DIRECTION('center_axis',(0.,0.,1.));
#10486=DIRECTION('ref_axis',(1.,0.,0.));
#10487=DIRECTION('center_axis',(0.,0.,1.));
#10488=DIRECTION('ref_axis',(1.,0.,0.));
#10489=DIRECTION('',(0.,0.,1.));
#10490=DIRECTION('center_axis',(0.,0.,-1.));
#10491=DIRECTION('ref_axis',(1.,0.,0.));
#10492=DIRECTION('center_axis',(0.,0.,1.));
#10493=DIRECTION('ref_axis',(-0.447213595499958,-0.894427190999916,0.));
#10494=DIRECTION('',(0.,0.,-1.));
#10495=DIRECTION('center_axis',(0.,0.,1.));
#10496=DIRECTION('ref_axis',(1.,0.,0.));
#10497=DIRECTION('',(0.,0.,1.));
#10498=DIRECTION('center_axis',(0.,0.,1.));
#10499=DIRECTION('ref_axis',(1.,0.,0.));
#10500=DIRECTION('center_axis',(0.,1.,0.));
#10501=DIRECTION('ref_axis',(1.,0.,0.));
#10502=DIRECTION('',(1.,0.,0.));
#10503=DIRECTION('',(0.,0.,-1.));
#10504=DIRECTION('',(-1.,0.,0.));
#10505=DIRECTION('center_axis',(0.,0.,-1.));
#10506=DIRECTION('ref_axis',(-1.,0.,0.));
#10507=DIRECTION('',(0.,1.,0.));
#10508=DIRECTION('',(-1.,0.,0.));
#10509=DIRECTION('',(0.,1.,0.));
#10510=DIRECTION('',(1.,0.,0.));
#10511=DIRECTION('',(0.,1.,0.));
#10512=DIRECTION('center_axis',(-1.,0.,0.));
#10513=DIRECTION('ref_axis',(0.,0.,1.));
#10514=DIRECTION('',(0.,1.,0.));
#10515=DIRECTION('',(0.,0.,1.));
#10516=DIRECTION('center_axis',(0.,1.,0.));
#10517=DIRECTION('ref_axis',(0.,0.,1.));
#10518=DIRECTION('',(1.,0.,0.));
#10519=DIRECTION('',(0.,0.,-1.));
#10520=DIRECTION('center_axis',(0.,0.,1.));
#10521=DIRECTION('ref_axis',(1.,0.,0.));
#10522=DIRECTION('',(0.,1.,0.));
#10523=DIRECTION('',(0.,1.,0.));
#10524=DIRECTION('center_axis',(-1.,0.,0.));
#10525=DIRECTION('ref_axis',(0.,0.,1.));
#10526=DIRECTION('',(0.,0.,-1.));
#10527=DIRECTION('',(0.,-1.,0.));
#10528=DIRECTION('center_axis',(1.,0.,0.));
#10529=DIRECTION('ref_axis',(0.,0.,-1.));
#10530=DIRECTION('',(0.,1.,0.));
#10531=DIRECTION('',(0.,0.,1.));
#10532=DIRECTION('center_axis',(0.,1.,0.));
#10533=DIRECTION('ref_axis',(1.,0.,0.));
#10534=DIRECTION('',(-1.,0.,0.));
#10535=DIRECTION('center_axis',(0.,1.,0.));
#10536=DIRECTION('ref_axis',(1.,0.,0.));
#10537=DIRECTION('center_axis',(0.,1.,0.));
#10538=DIRECTION('ref_axis',(1.,0.,0.));
#10539=DIRECTION('center_axis',(0.,1.,0.));
#10540=DIRECTION('ref_axis',(1.,0.,0.));
#10541=DIRECTION('center_axis',(0.,1.,0.));
#10542=DIRECTION('ref_axis',(1.,0.,0.));
#10543=DIRECTION('',(0.,1.,0.));
#10544=DIRECTION('center_axis',(0.,0.,-1.));
#10545=DIRECTION('ref_axis',(-1.,0.,0.));
#10546=DIRECTION('center_axis',(0.,0.,1.));
#10547=DIRECTION('ref_axis',(1.,0.,0.));
#10548=DIRECTION('center_axis',(0.,0.,1.));
#10549=DIRECTION('ref_axis',(1.,0.,0.));
#10550=DIRECTION('',(0.,0.,1.));
#10551=DIRECTION('center_axis',(0.,0.,-1.));
#10552=DIRECTION('ref_axis',(1.,0.,0.));
#10553=DIRECTION('center_axis',(-1.,0.,0.));
#10554=DIRECTION('ref_axis',(0.,0.,1.));
#10555=DIRECTION('',(0.,0.,-1.));
#10556=DIRECTION('',(0.,1.,0.));
#10557=DIRECTION('',(0.,0.,1.));
#10558=DIRECTION('',(0.,1.,0.));
#10559=DIRECTION('center_axis',(0.,0.,-1.));
#10560=DIRECTION('ref_axis',(-1.,0.,0.));
#10561=DIRECTION('',(1.,0.,0.));
#10562=DIRECTION('',(-1.,0.,0.));
#10563=DIRECTION('',(0.,1.,0.));
#10564=DIRECTION('center_axis',(1.,0.,0.));
#10565=DIRECTION('ref_axis',(0.,0.,-1.));
#10566=DIRECTION('',(0.,0.,1.));
#10567=DIRECTION('',(0.,0.,-1.));
#10568=DIRECTION('',(0.,1.,0.));
#10569=DIRECTION('center_axis',(0.,0.,1.));
#10570=DIRECTION('ref_axis',(1.,0.,0.));
#10571=DIRECTION('',(-1.,0.,0.));
#10572=DIRECTION('',(1.,0.,0.));
#10573=DIRECTION('center_axis',(0.,1.,0.));
#10574=DIRECTION('ref_axis',(0.,0.,1.));
#10575=DIRECTION('center_axis',(0.,1.,0.));
#10576=DIRECTION('ref_axis',(1.,0.,0.));
#10577=DIRECTION('center_axis',(0.,0.,1.));
#10578=DIRECTION('ref_axis',(1.,0.,0.));
#10579=DIRECTION('center_axis',(0.,0.,1.));
#10580=DIRECTION('ref_axis',(1.,0.,0.));
#10581=DIRECTION('',(0.,0.,1.));
#10582=DIRECTION('center_axis',(0.,0.,-1.));
#10583=DIRECTION('ref_axis',(1.,0.,0.));
#10584=DIRECTION('center_axis',(-1.,0.,0.));
#10585=DIRECTION('ref_axis',(0.,0.,1.));
#10586=DIRECTION('',(0.,0.,-1.));
#10587=DIRECTION('',(0.,1.,0.));
#10588=DIRECTION('',(0.,0.,1.));
#10589=DIRECTION('',(0.,1.,0.));
#10590=DIRECTION('center_axis',(0.,0.,-1.));
#10591=DIRECTION('ref_axis',(-1.,0.,0.));
#10592=DIRECTION('',(1.,0.,0.));
#10593=DIRECTION('',(-1.,0.,0.));
#10594=DIRECTION('',(0.,1.,0.));
#10595=DIRECTION('center_axis',(1.,0.,0.));
#10596=DIRECTION('ref_axis',(0.,0.,-1.));
#10597=DIRECTION('',(0.,0.,1.));
#10598=DIRECTION('',(0.,0.,-1.));
#10599=DIRECTION('',(0.,1.,0.));
#10600=DIRECTION('center_axis',(0.,0.,1.));
#10601=DIRECTION('ref_axis',(1.,0.,0.));
#10602=DIRECTION('',(-1.,0.,0.));
#10603=DIRECTION('',(1.,0.,0.));
#10604=DIRECTION('center_axis',(0.,1.,0.));
#10605=DIRECTION('ref_axis',(0.,0.,1.));
#10606=DIRECTION('center_axis',(0.,1.,0.));
#10607=DIRECTION('ref_axis',(1.,0.,0.));
#28032=CARTESIAN_POINT('',(0.,0.,0.));
#28033=CARTESIAN_POINT('Origin',(0.,-1.1,18.));
#28034=CARTESIAN_POINT('',(1.09971587239614,-1.,17.975));
#28035=CARTESIAN_POINT('',(-1.09971587239614,-1.,17.975));
#28036=CARTESIAN_POINT('Origin',(0.,-1.,18.));
#28037=CARTESIAN_POINT('',(1.09971587239614,1.,17.975));
#28038=CARTESIAN_POINT('',(1.09971587239614,-1.1,17.975));
#28039=CARTESIAN_POINT('',(-1.09971587239614,1.,17.975));
#28040=CARTESIAN_POINT('Origin',(0.,1.,18.));
#28041=CARTESIAN_POINT('',(-1.09971587239614,-1.1,17.975));
#28042=CARTESIAN_POINT('Origin',(0.,1.,18.));
#28043=CARTESIAN_POINT('',(1.99984374389601,1.,17.975));
#28044=CARTESIAN_POINT('',(2.,1.,17.975));
#28045=CARTESIAN_POINT('',(0.8,1.,16.1669697220177));
#28046=CARTESIAN_POINT('Origin',(0.,1.,18.));
#28047=CARTESIAN_POINT('',(0.8,1.,16.2));
#28048=CARTESIAN_POINT('',(0.8,1.,17.1));
#28049=CARTESIAN_POINT('',(-0.8,1.,16.2));
#28050=CARTESIAN_POINT('',(-0.4,1.,16.2));
#28051=CARTESIAN_POINT('',(-0.8,1.,16.1669697220177));
#28052=CARTESIAN_POINT('',(-0.8,1.,16.5));
#28053=CARTESIAN_POINT('',(-1.99984374389601,1.,17.975));
#28054=CARTESIAN_POINT('Origin',(0.,1.,18.));
#28055=CARTESIAN_POINT('',(2.,1.,17.975));
#28056=CARTESIAN_POINT('Origin',(4.,-1.1,17.975));
#28057=CARTESIAN_POINT('',(1.99984374389601,-1.,17.975));
#28058=CARTESIAN_POINT('',(2.,-1.,17.975));
#28059=CARTESIAN_POINT('',(1.99984374389601,-1.,17.975));
#28060=CARTESIAN_POINT('Origin',(-8.5,0.,14.9));
#28061=CARTESIAN_POINT('',(-9.71,-1.4818226269683E-16,15.));
#28062=CARTESIAN_POINT('Origin',(-8.5,0.,15.));
#28063=CARTESIAN_POINT('',(-9.71,1.4818226269683E-16,16.2));
#28064=CARTESIAN_POINT('',(-9.71,-1.4818226269683E-16,14.9));
#28065=CARTESIAN_POINT('Origin',(-8.5,0.,16.2));
#28066=CARTESIAN_POINT('Origin',(-8.5,0.,15.));
#28067=CARTESIAN_POINT('',(-6.9,1.2,16.2));
#28068=CARTESIAN_POINT('',(-6.9,1.2,15.));
#28069=CARTESIAN_POINT('',(-6.9,1.2,15.));
#28070=CARTESIAN_POINT('',(-8.5,2.,16.2));
#28071=CARTESIAN_POINT('Origin',(-8.5,0.,16.2));
#28072=CARTESIAN_POINT('',(-8.5,2.,15.));
#28073=CARTESIAN_POINT('',(-8.5,2.,15.));
#28074=CARTESIAN_POINT('Origin',(-8.5,0.,15.));
#28075=CARTESIAN_POINT('Origin',(-4.25,1.2,15.6));
#28076=CARTESIAN_POINT('',(-0.8,1.2,15.));
#28077=CARTESIAN_POINT('',(-8.5,1.2,15.));
#28078=CARTESIAN_POINT('',(-0.8,1.2,16.2));
#28079=CARTESIAN_POINT('',(-0.8,1.2,15.3));
#28080=CARTESIAN_POINT('',(0.,1.2,16.2));
#28081=CARTESIAN_POINT('Origin',(0.8,-1.,15.));
#28082=CARTESIAN_POINT('',(-8.5,3.2,15.));
#28083=CARTESIAN_POINT('',(-8.5,1.2,15.));
#28084=CARTESIAN_POINT('',(0.8,3.2,15.));
#28085=CARTESIAN_POINT('',(-0.8,3.2,15.));
#28086=CARTESIAN_POINT('',(0.8,-1.,15.));
#28087=CARTESIAN_POINT('',(0.8,-1.,15.));
#28088=CARTESIAN_POINT('',(-0.8,-1.,15.));
#28089=CARTESIAN_POINT('',(-0.8,-1.,15.));
#28090=CARTESIAN_POINT('',(-0.8,-1.,15.));
#28091=CARTESIAN_POINT('Origin',(-8.5,1.2,15.));
#28092=CARTESIAN_POINT('',(-8.5,3.2,16.2));
#28093=CARTESIAN_POINT('',(-8.5,1.2,16.2));
#28094=CARTESIAN_POINT('',(-8.5,3.2,16.2));
#28095=CARTESIAN_POINT('Origin',(0.,3.2,15.6));
#28096=CARTESIAN_POINT('',(0.8,3.2,16.2));
#28097=CARTESIAN_POINT('',(0.,3.2,16.2));
#28098=CARTESIAN_POINT('',(0.8,3.2,15.));
#28099=CARTESIAN_POINT('Origin',(-0.8,-1.,16.2));
#28100=CARTESIAN_POINT('',(-0.8,-1.,16.2));
#28101=CARTESIAN_POINT('',(0.8,-1.,16.2));
#28102=CARTESIAN_POINT('Origin',(-0.8,-1.,15.));
#28103=CARTESIAN_POINT('',(-0.8,-1.,16.1669697220177));
#28104=CARTESIAN_POINT('',(-0.8,-1.,16.2));
#28105=CARTESIAN_POINT('',(-0.8,-1.,16.1669697220177));
#28106=CARTESIAN_POINT('Origin',(0.8,-1.,16.2));
#28107=CARTESIAN_POINT('',(0.8,-1.,16.1669697220177));
#28108=CARTESIAN_POINT('',(0.8,-1.,16.1669697220177));
#28109=CARTESIAN_POINT('',(0.8,-1.,15.));
#28110=CARTESIAN_POINT('Origin',(0.,-1.,18.));
#28111=CARTESIAN_POINT('',(-1.99984374389601,-1.,17.975));
#28112=CARTESIAN_POINT('',(2.,-1.,17.975));
#28113=CARTESIAN_POINT('Origin',(0.,-1.,18.));
#28114=CARTESIAN_POINT('Origin',(0.,-1.,18.));
#28115=CARTESIAN_POINT('Origin',(0.,-1.,18.));
#28116=CARTESIAN_POINT('Origin',(0.,-1.,18.));
#28117=CARTESIAN_POINT('',(-1.99984374389601,-1.,17.975));
#28118=CARTESIAN_POINT('Origin',(4.,-1.1,17.975));
#28119=CARTESIAN_POINT('Origin',(-3.,0.,16.7));
#28120=CARTESIAN_POINT('',(-3.425,-5.20474889637625E-17,16.8));
#28121=CARTESIAN_POINT('Origin',(-3.,0.,16.8));
#28122=CARTESIAN_POINT('',(-3.425,5.20474889637625E-17,17.975));
#28123=CARTESIAN_POINT('',(-3.425,-5.20474889637625E-17,16.7));
#28124=CARTESIAN_POINT('Origin',(-3.,0.,17.975));
#28125=CARTESIAN_POINT('Origin',(-4.,-1.,16.8));
#28126=CARTESIAN_POINT('',(-4.,-1.,17.975));
#28127=CARTESIAN_POINT('',(-4.,-1.,16.8));
#28128=CARTESIAN_POINT('',(-4.,-1.,17.975));
#28129=CARTESIAN_POINT('',(-4.,1.,17.975));
#28130=CARTESIAN_POINT('',(-4.,-1.,17.975));
#28131=CARTESIAN_POINT('',(-4.,1.,16.8));
#28132=CARTESIAN_POINT('',(-4.,1.,17.975));
#28133=CARTESIAN_POINT('',(-4.,-1.,16.8));
#28134=CARTESIAN_POINT('Origin',(-2.,-1.,16.8));
#28135=CARTESIAN_POINT('',(-2.,-1.,16.8));
#28136=CARTESIAN_POINT('',(-4.,-1.,16.8));
#28137=CARTESIAN_POINT('',(-2.,1.,16.8));
#28138=CARTESIAN_POINT('',(-4.,1.,16.8));
#28139=CARTESIAN_POINT('',(-2.,-1.,16.8));
#28140=CARTESIAN_POINT('Origin',(-2.,-1.,17.975));
#28141=CARTESIAN_POINT('',(-2.,-1.,17.975));
#28142=CARTESIAN_POINT('',(-2.,-1.,16.8));
#28143=CARTESIAN_POINT('',(-2.,1.,17.975));
#28144=CARTESIAN_POINT('',(-2.,1.,16.8));
#28145=CARTESIAN_POINT('',(-2.,-1.,17.975));
#28146=CARTESIAN_POINT('Origin',(-4.,-1.,17.975));
#28147=CARTESIAN_POINT('',(-2.,-1.,17.975));
#28148=CARTESIAN_POINT('',(-2.,1.,17.975));
#28149=CARTESIAN_POINT('Origin',(-3.,1.,17.3875));
#28150=CARTESIAN_POINT('Origin',(-3.,-1.,17.3875));
#28151=CARTESIAN_POINT('Origin',(3.,0.,16.7));
#28152=CARTESIAN_POINT('',(2.575,-5.20474889637625E-17,16.8));
#28153=CARTESIAN_POINT('Origin',(3.,0.,16.8));
#28154=CARTESIAN_POINT('',(2.575,5.20474889637625E-17,17.975));
#28155=CARTESIAN_POINT('',(2.575,-5.20474889637625E-17,16.7));
#28156=CARTESIAN_POINT('Origin',(3.,0.,17.975));
#28157=CARTESIAN_POINT('Origin',(2.,-1.,16.8));
#28158=CARTESIAN_POINT('',(2.,-1.,17.975));
#28159=CARTESIAN_POINT('',(2.,-1.,16.8));
#28160=CARTESIAN_POINT('',(2.,-1.,17.975));
#28161=CARTESIAN_POINT('',(2.,1.,17.975));
#28162=CARTESIAN_POINT('',(2.,-1.,17.975));
#28163=CARTESIAN_POINT('',(2.,1.,16.8));
#28164=CARTESIAN_POINT('',(2.,1.,17.975));
#28165=CARTESIAN_POINT('',(2.,-1.,16.8));
#28166=CARTESIAN_POINT('Origin',(4.,-1.,16.8));
#28167=CARTESIAN_POINT('',(4.,-1.,16.8));
#28168=CARTESIAN_POINT('',(2.,-1.,16.8));
#28169=CARTESIAN_POINT('',(4.,1.,16.8));
#28170=CARTESIAN_POINT('',(2.,1.,16.8));
#28171=CARTESIAN_POINT('',(4.,-1.,16.8));
#28172=CARTESIAN_POINT('Origin',(4.,-1.,17.975));
#28173=CARTESIAN_POINT('',(4.,-1.,17.975));
#28174=CARTESIAN_POINT('',(4.,-1.,16.8));
#28175=CARTESIAN_POINT('',(4.,1.,17.975));
#28176=CARTESIAN_POINT('',(4.,1.,16.8));
#28177=CARTESIAN_POINT('',(4.,-1.,17.975));
#28178=CARTESIAN_POINT('Origin',(2.,-1.,17.975));
#28179=CARTESIAN_POINT('',(4.,-1.,17.975));
#28180=CARTESIAN_POINT('',(4.,1.,17.975));
#28181=CARTESIAN_POINT('Origin',(3.,1.,17.3875));
#28182=CARTESIAN_POINT('Origin',(3.,-1.,17.3875));
#34382=UNCERTAINTY_MEASURE_WITH_UNIT(LENGTH_MEASURE(0.001),#34434,
'DISTANCE_ACCURACY_VALUE',
'Maximum model space distance between geometric entities at asserted c
onnectivities');
#34404=UNCERTAINTY_MEASURE_WITH_UNIT(LENGTH_MEASURE(0.001),#34434,
'DISTANCE_ACCURACY_VALUE',
'Maximum model space distance between geometric entities at asserted c
onnectivities');
#34411=(
GEOMETRIC_REPRESENTATION_CONTEXT(3)
GLOBAL_UNCERTAINTY_ASSIGNED_CONTEXT((#34382))
GLOBAL_UNIT_ASSIGNED_CONTEXT((#34434,#34436,#34437))
REPRESENTATION_CONTEXT('','3D')
);
#34433=(
GEOMETRIC_REPRESENTATION_CONTEXT(3)
GLOBAL_UNCERTAINTY_ASSIGNED_CONTEXT((#34404))
GLOBAL_UNIT_ASSIGNED_CONTEXT((#34434,#34436,#34437))
REPRESENTATION_CONTEXT('','3D')
);
#34434=(
LENGTH_UNIT()
NAMED_UNIT(*)
SI_UNIT(.CENTI.,.METRE.)
);
#34436=(
NAMED_UNIT(*)
PLANE_ANGLE_UNIT()
SI_UNIT($,.RADIAN.)
);
#34437=(
NAMED_UNIT(*)
SI_UNIT($,.STERADIAN.)
SOLID_ANGLE_UNIT()
);
#34444=SHAPE_DEFINITION_REPRESENTATION(#34472,#34543);
#34472=PRODUCT_DEFINITION_SHAPE('',$,#34572);
#34543=SHAPE_REPRESENTATION('',(#9303),#34411);
#34565=PRODUCT_DEFINITION_CONTEXT('part definition',#34651,'design');
#34572=PRODUCT_DEFINITION('Lower 20 mm clamp','Lower 20 mm clamp',#34600,
#34565);
#34600=PRODUCT_DEFINITION_FORMATION('',$,#34659);
#34651=APPLICATION_CONTEXT(
'Core Data for Automotive Mechanical Design Process');
#34652=PRODUCT_CONTEXT('part definition',#34651,'mechanical');
#34659=PRODUCT('Lower 20 mm clamp','Lower 20 mm clamp',
'Lower 20 mm clamp',(#34652));
#34723=COLOUR_RGB('Light Blue',0.38,0.62,0.78);
#34724=FILL_AREA_STYLE_COLOUR('',#34723);
#34725=FILL_AREA_STYLE('',(#34724));
#34726=SURFACE_STYLE_FILL_AREA(#34725);
#34727=SURFACE_SIDE_STYLE('',(#34726));
#34728=SURFACE_STYLE_USAGE(.BOTH.,#34727);
#34729=PRESENTATION_STYLE_ASSIGNMENT((#34728));
ENDSEC;
END-ISO-10303-21;
